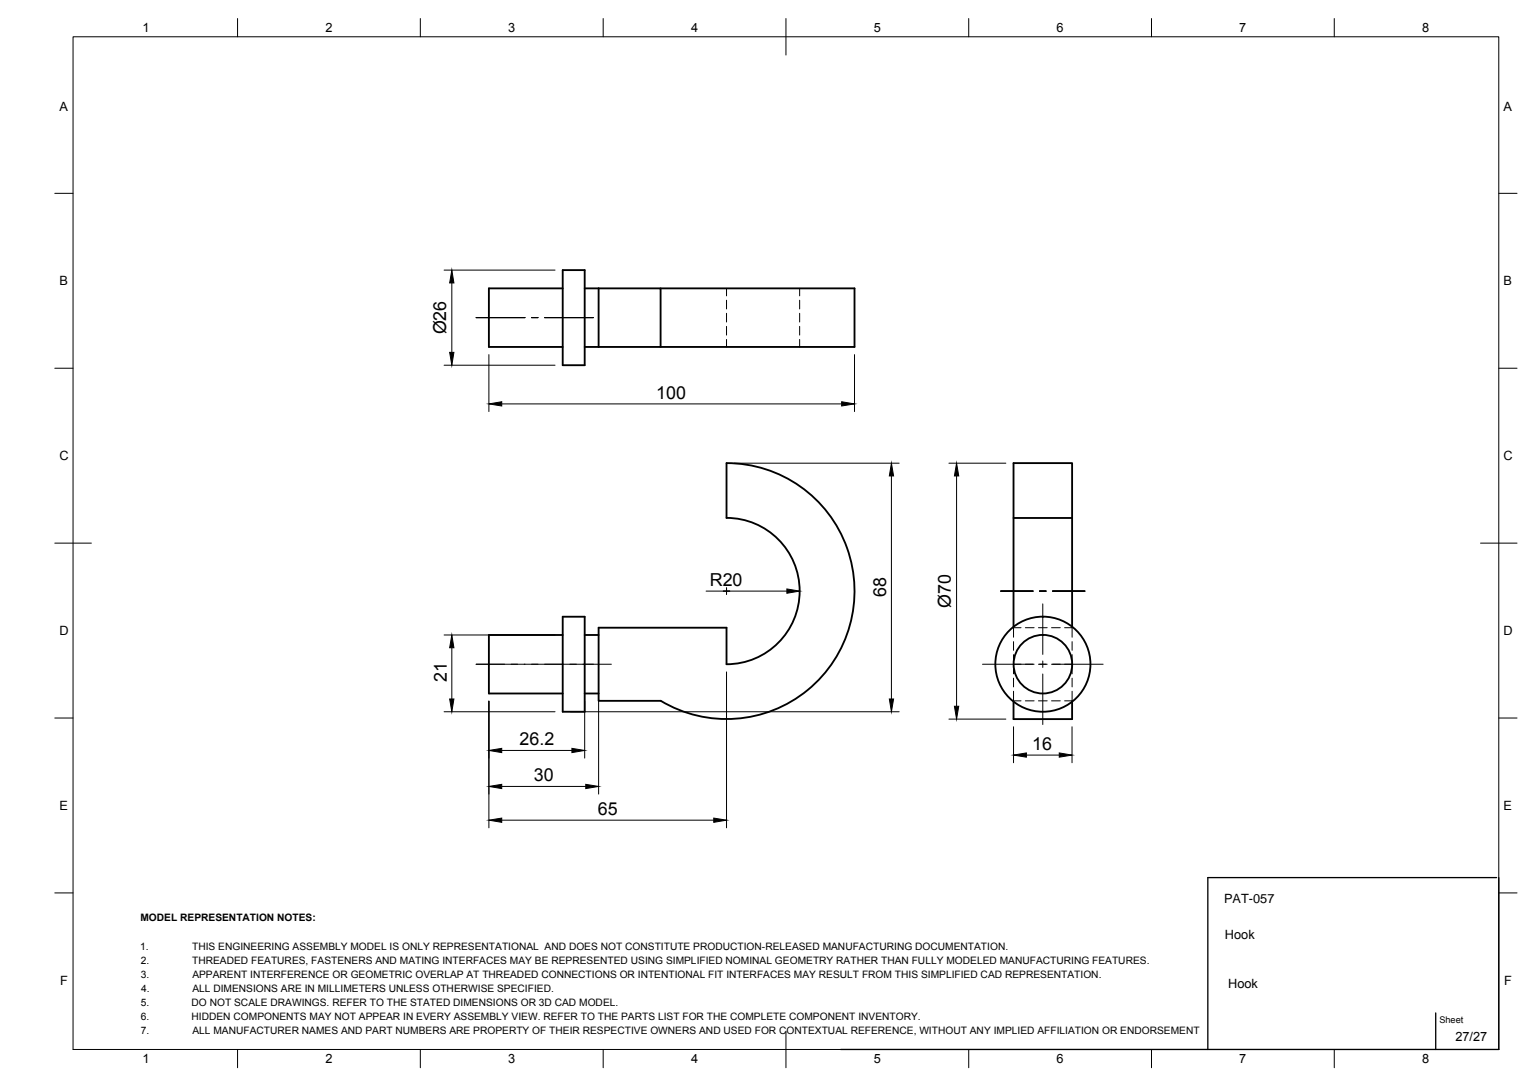
ISO-10303-21;
HEADER;
/* Generated by software containing ST-Developer
 * from STEP Tools, Inc. (www.steptools.com) 
 */

FILE_DESCRIPTION(
/* description */ ('Bearing-mounted hook block'),
/* implementation_level */ '2;1');

FILE_NAME(
/* name */ 'Hook.step',
/* time_stamp */ '2026-10-28T22:30:11-07:00',
/* author */ (''),
/* organization */ (''),
/* preprocessor_version */ 'ST-DEVELOPER v20.2',
/* originating_system */ 'Autodesk Translation Framework v15.17.0.0',
/* authorisation */ '');

FILE_SCHEMA (('AUTOMOTIVE_DESIGN { 1 0 10303 214 3 1 1 }'));
ENDSEC;

DATA;
#10=MECHANICAL_DESIGN_GEOMETRIC_PRESENTATION_REPRESENTATION('',(#352),#7609);
#296=SHAPE_REPRESENTATION_RELATIONSHIP('SRR','None',#7746,#320);
#320=ADVANCED_BREP_SHAPE_REPRESENTATION('',(#381),#7606);
#352=STYLED_ITEM('',(#7917),#381);
#381=MANIFOLD_SOLID_BREP('Body1',#3951);
#571=LINE('',#7423,#801);
#572=LINE('',#7426,#802);
#573=LINE('',#7435,#803);
#574=LINE('',#7439,#804);
#575=LINE('',#7441,#805);
#576=LINE('',#7442,#806);
#577=LINE('',#7445,#807);
#578=LINE('',#7447,#808);
#579=LINE('',#7448,#809);
#580=LINE('',#7452,#810);
#581=LINE('',#7453,#811);
#582=LINE('',#7454,#812);
#583=LINE('',#7458,#813);
#584=LINE('',#7460,#814);
#585=LINE('',#7462,#815);
#586=LINE('',#7463,#816);
#587=LINE('',#7465,#817);
#588=LINE('',#7469,#818);
#589=LINE('',#7474,#819);
#590=LINE('',#7476,#820);
#591=LINE('',#7479,#821);
#592=LINE('',#7482,#822);
#801=VECTOR('',#5924,1.3);
#802=VECTOR('',#5927,0.8);
#803=VECTOR('',#5938,0.8);
#804=VECTOR('',#5943,1.);
#805=VECTOR('',#5944,1.);
#806=VECTOR('',#5945,1.);
#807=VECTOR('',#5948,1.);
#808=VECTOR('',#5949,1.);
#809=VECTOR('',#5950,1.);
#810=VECTOR('',#5953,1.);
#811=VECTOR('',#5954,1.);
#812=VECTOR('',#5955,1.);
#813=VECTOR('',#5958,1.);
#814=VECTOR('',#5959,1.);
#815=VECTOR('',#5960,1.);
#816=VECTOR('',#5961,1.);
#817=VECTOR('',#5964,1.);
#818=VECTOR('',#5967,1.);
#819=VECTOR('',#5974,1.);
#820=VECTOR('',#5977,1.);
#821=VECTOR('',#5980,1.);
#822=VECTOR('',#5985,1.);
#913=CYLINDRICAL_SURFACE('',#4708,1.3);
#914=CYLINDRICAL_SURFACE('',#4709,0.8);
#915=CYLINDRICAL_SURFACE('',#4713,0.8);
#916=CYLINDRICAL_SURFACE('',#4723,2.);
#917=CYLINDRICAL_SURFACE('',#4729,3.5);
#995=FACE_BOUND('',#1519,.T.);
#996=FACE_BOUND('',#1521,.T.);
#1208=FACE_OUTER_BOUND('',#1518,.T.);
#1209=FACE_OUTER_BOUND('',#1520,.T.);
#1210=FACE_OUTER_BOUND('',#1522,.T.);
#1211=FACE_OUTER_BOUND('',#1523,.T.);
#1212=FACE_OUTER_BOUND('',#1524,.T.);
#1213=FACE_OUTER_BOUND('',#1525,.T.);
#1214=FACE_OUTER_BOUND('',#1526,.T.);
#1215=FACE_OUTER_BOUND('',#1527,.T.);
#1216=FACE_OUTER_BOUND('',#1528,.T.);
#1217=FACE_OUTER_BOUND('',#1529,.T.);
#1218=FACE_OUTER_BOUND('',#1530,.T.);
#1219=FACE_OUTER_BOUND('',#1531,.T.);
#1220=FACE_OUTER_BOUND('',#1532,.T.);
#1221=FACE_OUTER_BOUND('',#1533,.T.);
#1222=FACE_OUTER_BOUND('',#1534,.T.);
#1223=FACE_OUTER_BOUND('',#1535,.T.);
#1518=EDGE_LOOP('',(#3438));
#1519=EDGE_LOOP('',(#3439));
#1520=EDGE_LOOP('',(#3440));
#1521=EDGE_LOOP('',(#3441));
#1522=EDGE_LOOP('',(#3442,#3443,#3444,#3445));
#1523=EDGE_LOOP('',(#3446,#3447,#3448,#3449,#3450,#3451));
#1524=EDGE_LOOP('',(#3452,#3453,#3454,#3455));
#1525=EDGE_LOOP('',(#3456));
#1526=EDGE_LOOP('',(#3457,#3458,#3459,#3460));
#1527=EDGE_LOOP('',(#3461,#3462,#3463,#3464,#3465));
#1528=EDGE_LOOP('',(#3466,#3467,#3468,#3469));
#1529=EDGE_LOOP('',(#3470,#3471,#3472,#3473));
#1530=EDGE_LOOP('',(#3474,#3475,#3476,#3477,#3478,#3479,#3480,#3481));
#1531=EDGE_LOOP('',(#3482,#3483,#3484,#3485));
#1532=EDGE_LOOP('',(#3486,#3487,#3488,#3489,#3490,#3491,#3492,#3493));
#1533=EDGE_LOOP('',(#3494,#3495,#3496,#3497));
#1534=EDGE_LOOP('',(#3498,#3499,#3500,#3501));
#1535=EDGE_LOOP('',(#3502,#3503,#3504,#3505));
#1760=CIRCLE('',#4703,1.3);
#1761=CIRCLE('',#4704,0.8);
#1762=CIRCLE('',#4706,1.3);
#1763=CIRCLE('',#4707,0.8);
#1764=CIRCLE('',#4710,0.8);
#1765=CIRCLE('',#4711,0.8);
#1766=CIRCLE('',#4712,0.8);
#1767=CIRCLE('',#4714,0.8);
#1768=CIRCLE('',#4721,2.);
#1769=CIRCLE('',#4722,3.5);
#1770=CIRCLE('',#4724,2.);
#1771=CIRCLE('',#4726,3.5);
#2065=VERTEX_POINT('',#7413);
#2066=VERTEX_POINT('',#7415);
#2067=VERTEX_POINT('',#7418);
#2068=VERTEX_POINT('',#7420);
#2069=VERTEX_POINT('',#7425);
#2070=VERTEX_POINT('',#7427);
#2071=VERTEX_POINT('',#7429);
#2072=VERTEX_POINT('',#7433);
#2073=VERTEX_POINT('',#7438);
#2074=VERTEX_POINT('',#7440);
#2075=VERTEX_POINT('',#7444);
#2076=VERTEX_POINT('',#7446);
#2077=VERTEX_POINT('',#7450);
#2078=VERTEX_POINT('',#7451);
#2079=VERTEX_POINT('',#7456);
#2080=VERTEX_POINT('',#7457);
#2081=VERTEX_POINT('',#7459);
#2082=VERTEX_POINT('',#7461);
#2083=VERTEX_POINT('',#7466);
#2084=VERTEX_POINT('',#7468);
#2085=VERTEX_POINT('',#7472);
#2086=VERTEX_POINT('',#7477);
#2529=EDGE_CURVE('',#2065,#2065,#1760,.T.);
#2530=EDGE_CURVE('',#2066,#2066,#1761,.T.);
#2531=EDGE_CURVE('',#2067,#2067,#1762,.T.);
#2532=EDGE_CURVE('',#2068,#2068,#1763,.T.);
#2533=EDGE_CURVE('',#2065,#2067,#571,.T.);
#2534=EDGE_CURVE('',#2068,#2069,#572,.T.);
#2535=EDGE_CURVE('',#2070,#2069,#1764,.T.);
#2536=EDGE_CURVE('',#2071,#2070,#1765,.T.);
#2537=EDGE_CURVE('',#2069,#2071,#1766,.T.);
#2538=EDGE_CURVE('',#2072,#2072,#1767,.T.);
#2539=EDGE_CURVE('',#2072,#2066,#573,.T.);
#2540=EDGE_CURVE('',#2073,#2070,#574,.T.);
#2541=EDGE_CURVE('',#2073,#2074,#575,.T.);
#2542=EDGE_CURVE('',#2071,#2074,#576,.T.);
#2543=EDGE_CURVE('',#2075,#2071,#577,.T.);
#2544=EDGE_CURVE('',#2076,#2075,#578,.T.);
#2545=EDGE_CURVE('',#2070,#2076,#579,.T.);
#2546=EDGE_CURVE('',#2077,#2078,#580,.T.);
#2547=EDGE_CURVE('',#2076,#2077,#581,.T.);
#2548=EDGE_CURVE('',#2078,#2075,#582,.T.);
#2549=EDGE_CURVE('',#2079,#2080,#583,.T.);
#2550=EDGE_CURVE('',#2081,#2079,#584,.T.);
#2551=EDGE_CURVE('',#2082,#2081,#585,.T.);
#2552=EDGE_CURVE('',#2080,#2082,#586,.T.);
#2553=EDGE_CURVE('',#2074,#2081,#587,.T.);
#2554=EDGE_CURVE('',#2079,#2083,#1768,.T.);
#2555=EDGE_CURVE('',#2083,#2084,#588,.T.);
#2556=EDGE_CURVE('',#2084,#2078,#1769,.T.);
#2557=EDGE_CURVE('',#2080,#2085,#1770,.T.);
#2558=EDGE_CURVE('',#2085,#2083,#589,.T.);
#2559=EDGE_CURVE('',#2082,#2073,#590,.T.);
#2560=EDGE_CURVE('',#2086,#2077,#1771,.T.);
#2561=EDGE_CURVE('',#2086,#2085,#591,.T.);
#2562=EDGE_CURVE('',#2084,#2086,#592,.T.);
#3438=ORIENTED_EDGE('',*,*,#2529,.T.);
#3439=ORIENTED_EDGE('',*,*,#2530,.F.);
#3440=ORIENTED_EDGE('',*,*,#2531,.F.);
#3441=ORIENTED_EDGE('',*,*,#2532,.F.);
#3442=ORIENTED_EDGE('',*,*,#2529,.F.);
#3443=ORIENTED_EDGE('',*,*,#2533,.T.);
#3444=ORIENTED_EDGE('',*,*,#2531,.T.);
#3445=ORIENTED_EDGE('',*,*,#2533,.F.);
#3446=ORIENTED_EDGE('',*,*,#2532,.T.);
#3447=ORIENTED_EDGE('',*,*,#2534,.T.);
#3448=ORIENTED_EDGE('',*,*,#2535,.F.);
#3449=ORIENTED_EDGE('',*,*,#2536,.F.);
#3450=ORIENTED_EDGE('',*,*,#2537,.F.);
#3451=ORIENTED_EDGE('',*,*,#2534,.F.);
#3452=ORIENTED_EDGE('',*,*,#2538,.F.);
#3453=ORIENTED_EDGE('',*,*,#2539,.T.);
#3454=ORIENTED_EDGE('',*,*,#2530,.T.);
#3455=ORIENTED_EDGE('',*,*,#2539,.F.);
#3456=ORIENTED_EDGE('',*,*,#2538,.T.);
#3457=ORIENTED_EDGE('',*,*,#2536,.T.);
#3458=ORIENTED_EDGE('',*,*,#2540,.F.);
#3459=ORIENTED_EDGE('',*,*,#2541,.T.);
#3460=ORIENTED_EDGE('',*,*,#2542,.F.);
#3461=ORIENTED_EDGE('',*,*,#2535,.T.);
#3462=ORIENTED_EDGE('',*,*,#2537,.T.);
#3463=ORIENTED_EDGE('',*,*,#2543,.F.);
#3464=ORIENTED_EDGE('',*,*,#2544,.F.);
#3465=ORIENTED_EDGE('',*,*,#2545,.F.);
#3466=ORIENTED_EDGE('',*,*,#2546,.F.);
#3467=ORIENTED_EDGE('',*,*,#2547,.F.);
#3468=ORIENTED_EDGE('',*,*,#2544,.T.);
#3469=ORIENTED_EDGE('',*,*,#2548,.F.);
#3470=ORIENTED_EDGE('',*,*,#2549,.F.);
#3471=ORIENTED_EDGE('',*,*,#2550,.F.);
#3472=ORIENTED_EDGE('',*,*,#2551,.F.);
#3473=ORIENTED_EDGE('',*,*,#2552,.F.);
#3474=ORIENTED_EDGE('',*,*,#2553,.T.);
#3475=ORIENTED_EDGE('',*,*,#2550,.T.);
#3476=ORIENTED_EDGE('',*,*,#2554,.T.);
#3477=ORIENTED_EDGE('',*,*,#2555,.T.);
#3478=ORIENTED_EDGE('',*,*,#2556,.T.);
#3479=ORIENTED_EDGE('',*,*,#2548,.T.);
#3480=ORIENTED_EDGE('',*,*,#2543,.T.);
#3481=ORIENTED_EDGE('',*,*,#2542,.T.);
#3482=ORIENTED_EDGE('',*,*,#2549,.T.);
#3483=ORIENTED_EDGE('',*,*,#2557,.T.);
#3484=ORIENTED_EDGE('',*,*,#2558,.T.);
#3485=ORIENTED_EDGE('',*,*,#2554,.F.);
#3486=ORIENTED_EDGE('',*,*,#2559,.T.);
#3487=ORIENTED_EDGE('',*,*,#2540,.T.);
#3488=ORIENTED_EDGE('',*,*,#2545,.T.);
#3489=ORIENTED_EDGE('',*,*,#2547,.T.);
#3490=ORIENTED_EDGE('',*,*,#2560,.F.);
#3491=ORIENTED_EDGE('',*,*,#2561,.T.);
#3492=ORIENTED_EDGE('',*,*,#2557,.F.);
#3493=ORIENTED_EDGE('',*,*,#2552,.T.);
#3494=ORIENTED_EDGE('',*,*,#2559,.F.);
#3495=ORIENTED_EDGE('',*,*,#2551,.T.);
#3496=ORIENTED_EDGE('',*,*,#2553,.F.);
#3497=ORIENTED_EDGE('',*,*,#2541,.F.);
#3498=ORIENTED_EDGE('',*,*,#2562,.F.);
#3499=ORIENTED_EDGE('',*,*,#2555,.F.);
#3500=ORIENTED_EDGE('',*,*,#2558,.F.);
#3501=ORIENTED_EDGE('',*,*,#2561,.F.);
#3502=ORIENTED_EDGE('',*,*,#2546,.T.);
#3503=ORIENTED_EDGE('',*,*,#2556,.F.);
#3504=ORIENTED_EDGE('',*,*,#2562,.T.);
#3505=ORIENTED_EDGE('',*,*,#2560,.T.);
#3662=PLANE('',#4702);
#3663=PLANE('',#4705);
#3664=PLANE('',#4715);
#3665=PLANE('',#4716);
#3666=PLANE('',#4717);
#3667=PLANE('',#4718);
#3668=PLANE('',#4719);
#3669=PLANE('',#4720);
#3670=PLANE('',#4725);
#3671=PLANE('',#4727);
#3672=PLANE('',#4728);
#3890=ADVANCED_FACE('',(#1208,#995),#3662,.T.);
#3891=ADVANCED_FACE('',(#1209,#996),#3663,.F.);
#3892=ADVANCED_FACE('',(#1210),#913,.T.);
#3893=ADVANCED_FACE('',(#1211),#914,.T.);
#3894=ADVANCED_FACE('',(#1212),#915,.T.);
#3895=ADVANCED_FACE('',(#1213),#3664,.T.);
#3896=ADVANCED_FACE('',(#1214),#3665,.T.);
#3897=ADVANCED_FACE('',(#1215),#3666,.T.);
#3898=ADVANCED_FACE('',(#1216),#3667,.T.);
#3899=ADVANCED_FACE('',(#1217),#3668,.T.);
#3900=ADVANCED_FACE('',(#1218),#3669,.T.);
#3901=ADVANCED_FACE('',(#1219),#916,.F.);
#3902=ADVANCED_FACE('',(#1220),#3670,.F.);
#3903=ADVANCED_FACE('',(#1221),#3671,.F.);
#3904=ADVANCED_FACE('',(#1222),#3672,.F.);
#3905=ADVANCED_FACE('',(#1223),#917,.T.);
#3951=CLOSED_SHELL('',(#3890,#3891,#3892,#3893,#3894,#3895,#3896,#3897,
#3898,#3899,#3900,#3901,#3902,#3903,#3904,#3905));
#4701=AXIS2_PLACEMENT_3D('',#7411,#5908,#5909);
#4702=AXIS2_PLACEMENT_3D('',#7412,#5910,#5911);
#4703=AXIS2_PLACEMENT_3D('',#7414,#5912,#5913);
#4704=AXIS2_PLACEMENT_3D('',#7416,#5914,#5915);
#4705=AXIS2_PLACEMENT_3D('',#7417,#5916,#5917);
#4706=AXIS2_PLACEMENT_3D('',#7419,#5918,#5919);
#4707=AXIS2_PLACEMENT_3D('',#7421,#5920,#5921);
#4708=AXIS2_PLACEMENT_3D('',#7422,#5922,#5923);
#4709=AXIS2_PLACEMENT_3D('',#7424,#5925,#5926);
#4710=AXIS2_PLACEMENT_3D('',#7428,#5928,#5929);
#4711=AXIS2_PLACEMENT_3D('',#7430,#5930,#5931);
#4712=AXIS2_PLACEMENT_3D('',#7431,#5932,#5933);
#4713=AXIS2_PLACEMENT_3D('',#7432,#5934,#5935);
#4714=AXIS2_PLACEMENT_3D('',#7434,#5936,#5937);
#4715=AXIS2_PLACEMENT_3D('',#7436,#5939,#5940);
#4716=AXIS2_PLACEMENT_3D('',#7437,#5941,#5942);
#4717=AXIS2_PLACEMENT_3D('',#7443,#5946,#5947);
#4718=AXIS2_PLACEMENT_3D('',#7449,#5951,#5952);
#4719=AXIS2_PLACEMENT_3D('',#7455,#5956,#5957);
#4720=AXIS2_PLACEMENT_3D('',#7464,#5962,#5963);
#4721=AXIS2_PLACEMENT_3D('',#7467,#5965,#5966);
#4722=AXIS2_PLACEMENT_3D('',#7470,#5968,#5969);
#4723=AXIS2_PLACEMENT_3D('',#7471,#5970,#5971);
#4724=AXIS2_PLACEMENT_3D('',#7473,#5972,#5973);
#4725=AXIS2_PLACEMENT_3D('',#7475,#5975,#5976);
#4726=AXIS2_PLACEMENT_3D('',#7478,#5978,#5979);
#4727=AXIS2_PLACEMENT_3D('',#7480,#5981,#5982);
#4728=AXIS2_PLACEMENT_3D('',#7481,#5983,#5984);
#4729=AXIS2_PLACEMENT_3D('',#7483,#5986,#5987);
#5908=DIRECTION('axis',(0.,0.,1.));
#5909=DIRECTION('refdir',(1.,0.,0.));
#5910=DIRECTION('center_axis',(0.,0.,1.));
#5911=DIRECTION('ref_axis',(1.,0.,0.));
#5912=DIRECTION('center_axis',(0.,0.,1.));
#5913=DIRECTION('ref_axis',(1.,0.,0.));
#5914=DIRECTION('center_axis',(0.,0.,1.));
#5915=DIRECTION('ref_axis',(1.,0.,0.));
#5916=DIRECTION('center_axis',(0.,0.,1.));
#5917=DIRECTION('ref_axis',(1.,0.,0.));
#5918=DIRECTION('center_axis',(0.,0.,1.));
#5919=DIRECTION('ref_axis',(1.,0.,0.));
#5920=DIRECTION('center_axis',(0.,0.,-1.));
#5921=DIRECTION('ref_axis',(1.,0.,0.));
#5922=DIRECTION('center_axis',(0.,0.,1.));
#5923=DIRECTION('ref_axis',(1.,0.,0.));
#5924=DIRECTION('',(0.,0.,-1.));
#5925=DIRECTION('center_axis',(0.,0.,1.));
#5926=DIRECTION('ref_axis',(1.,0.,0.));
#5927=DIRECTION('',(0.,0.,-1.));
#5928=DIRECTION('center_axis',(0.,0.,-1.));
#5929=DIRECTION('ref_axis',(1.,0.,0.));
#5930=DIRECTION('center_axis',(0.,0.,-1.));
#5931=DIRECTION('ref_axis',(1.,0.,0.));
#5932=DIRECTION('center_axis',(0.,0.,-1.));
#5933=DIRECTION('ref_axis',(1.,0.,0.));
#5934=DIRECTION('center_axis',(0.,0.,1.));
#5935=DIRECTION('ref_axis',(1.,0.,0.));
#5936=DIRECTION('center_axis',(0.,0.,1.));
#5937=DIRECTION('ref_axis',(1.,0.,0.));
#5938=DIRECTION('',(0.,0.,-1.));
#5939=DIRECTION('center_axis',(0.,0.,1.));
#5940=DIRECTION('ref_axis',(1.,0.,0.));
#5941=DIRECTION('center_axis',(0.,0.,1.));
#5942=DIRECTION('ref_axis',(1.,0.,0.));
#5943=DIRECTION('',(-1.,0.,0.));
#5944=DIRECTION('',(0.,1.,0.));
#5945=DIRECTION('',(1.,0.,0.));
#5946=DIRECTION('center_axis',(0.,0.,1.));
#5947=DIRECTION('ref_axis',(1.,0.,0.));
#5948=DIRECTION('',(1.,0.,0.));
#5949=DIRECTION('',(0.,1.,0.));
#5950=DIRECTION('',(-1.,0.,0.));
#5951=DIRECTION('center_axis',(-1.,0.,0.));
#5952=DIRECTION('ref_axis',(0.,0.,1.));
#5953=DIRECTION('',(0.,1.,0.));
#5954=DIRECTION('',(0.,0.,-1.));
#5955=DIRECTION('',(0.,0.,1.));
#5956=DIRECTION('center_axis',(0.,0.,-1.));
#5957=DIRECTION('ref_axis',(-1.,0.,0.));
#5958=DIRECTION('',(0.,-1.,0.));
#5959=DIRECTION('',(-1.,0.,0.));
#5960=DIRECTION('',(0.,1.,0.));
#5961=DIRECTION('',(1.,0.,0.));
#5962=DIRECTION('center_axis',(0.,1.,0.));
#5963=DIRECTION('ref_axis',(1.,0.,0.));
#5964=DIRECTION('',(0.,0.,-1.));
#5965=DIRECTION('center_axis',(0.,-1.,0.));
#5966=DIRECTION('ref_axis',(1.,0.,0.));
#5967=DIRECTION('',(1.,0.,0.));
#5968=DIRECTION('center_axis',(0.,1.,0.));
#5969=DIRECTION('ref_axis',(1.,0.,0.));
#5970=DIRECTION('center_axis',(0.,1.,0.));
#5971=DIRECTION('ref_axis',(1.,0.,0.));
#5972=DIRECTION('center_axis',(0.,-1.,0.));
#5973=DIRECTION('ref_axis',(1.,0.,0.));
#5974=DIRECTION('',(0.,1.,0.));
#5975=DIRECTION('center_axis',(0.,1.,0.));
#5976=DIRECTION('ref_axis',(1.,0.,0.));
#5977=DIRECTION('',(0.,0.,1.));
#5978=DIRECTION('center_axis',(0.,1.,0.));
#5979=DIRECTION('ref_axis',(1.,0.,0.));
#5980=DIRECTION('',(-1.,0.,0.));
#5981=DIRECTION('center_axis',(-1.,0.,0.));
#5982=DIRECTION('ref_axis',(0.,0.,1.));
#5983=DIRECTION('center_axis',(0.,0.,-1.));
#5984=DIRECTION('ref_axis',(-1.,0.,0.));
#5985=DIRECTION('',(0.,-1.,0.));
#5986=DIRECTION('center_axis',(0.,1.,0.));
#5987=DIRECTION('ref_axis',(-0.267261241912424,0.,-0.963624111659432));
#7411=CARTESIAN_POINT('',(0.,0.,0.));
#7412=CARTESIAN_POINT('Origin',(0.,0.,4.48));
#7413=CARTESIAN_POINT('',(-1.3,-1.59204083889156E-16,4.48));
#7414=CARTESIAN_POINT('Origin',(0.,0.,4.48));
#7415=CARTESIAN_POINT('',(-0.8,-9.79717439317883E-17,4.48));
#7416=CARTESIAN_POINT('Origin',(0.,0.,4.48));
#7417=CARTESIAN_POINT('Origin',(0.,0.,3.88));
#7418=CARTESIAN_POINT('',(-1.3,-1.59204083889156E-16,3.88));
#7419=CARTESIAN_POINT('Origin',(0.,0.,3.88));
#7420=CARTESIAN_POINT('',(-0.8,9.79717439317883E-17,3.88));
#7421=CARTESIAN_POINT('Origin',(0.,0.,3.88));
#7422=CARTESIAN_POINT('Origin',(0.,0.,3.88));
#7423=CARTESIAN_POINT('',(-1.3,-1.59204083889156E-16,3.88));
#7424=CARTESIAN_POINT('Origin',(0.,0.,3.));
#7425=CARTESIAN_POINT('',(-0.8,-9.79717439317883E-17,3.5));
#7426=CARTESIAN_POINT('',(-0.8,-9.79717439317883E-17,3.));
#7427=CARTESIAN_POINT('',(0.,-0.8,3.5));
#7428=CARTESIAN_POINT('Origin',(0.,0.,3.5));
#7429=CARTESIAN_POINT('',(0.,0.8,3.5));
#7430=CARTESIAN_POINT('Origin',(0.,0.,3.5));
#7431=CARTESIAN_POINT('Origin',(0.,0.,3.5));
#7432=CARTESIAN_POINT('Origin',(0.,0.,3.));
#7433=CARTESIAN_POINT('',(-0.8,-9.79717439317883E-17,6.5));
#7434=CARTESIAN_POINT('Origin',(0.,0.,6.5));
#7435=CARTESIAN_POINT('',(-0.8,-9.79717439317883E-17,3.));
#7436=CARTESIAN_POINT('Origin',(0.,0.,6.5));
#7437=CARTESIAN_POINT('Origin',(-1.,-0.8,3.5));
#7438=CARTESIAN_POINT('',(1.,-0.8,3.5));
#7439=CARTESIAN_POINT('',(1.,-0.8,3.5));
#7440=CARTESIAN_POINT('',(1.,0.8,3.5));
#7441=CARTESIAN_POINT('',(1.,-0.8,3.5));
#7442=CARTESIAN_POINT('',(1.,0.8,3.5));
#7443=CARTESIAN_POINT('Origin',(-1.,-0.8,3.5));
#7444=CARTESIAN_POINT('',(-1.,0.8,3.5));
#7445=CARTESIAN_POINT('',(1.,0.8,3.5));
#7446=CARTESIAN_POINT('',(-1.,-0.8,3.5));
#7447=CARTESIAN_POINT('',(-1.,-0.8,3.5));
#7448=CARTESIAN_POINT('',(1.,-0.8,3.5));
#7449=CARTESIAN_POINT('Origin',(-1.,-0.8,0.));
#7450=CARTESIAN_POINT('',(-1.,-0.8,1.80277563773199));
#7451=CARTESIAN_POINT('',(-1.,0.8,1.80277563773199));
#7452=CARTESIAN_POINT('',(-1.,-0.8,1.80277563773199));
#7453=CARTESIAN_POINT('',(-1.,-0.8,3.5));
#7454=CARTESIAN_POINT('',(-1.,0.8,3.5));
#7455=CARTESIAN_POINT('Origin',(1.,-0.8,0.));
#7456=CARTESIAN_POINT('',(0.,0.8,0.));
#7457=CARTESIAN_POINT('',(0.,-0.8,0.));
#7458=CARTESIAN_POINT('',(0.,-0.8,0.));
#7459=CARTESIAN_POINT('',(1.,0.8,0.));
#7460=CARTESIAN_POINT('',(-1.,0.8,0.));
#7461=CARTESIAN_POINT('',(1.,-0.8,0.));
#7462=CARTESIAN_POINT('',(1.,-0.8,0.));
#7463=CARTESIAN_POINT('',(-1.,-0.8,0.));
#7464=CARTESIAN_POINT('Origin',(2.,0.8,0.));
#7465=CARTESIAN_POINT('',(1.,0.8,0.));
#7466=CARTESIAN_POINT('',(4.,0.8,0.));
#7467=CARTESIAN_POINT('Origin',(2.,0.8,0.));
#7468=CARTESIAN_POINT('',(5.5,0.8,0.));
#7469=CARTESIAN_POINT('',(4.,0.8,0.));
#7470=CARTESIAN_POINT('Origin',(2.,0.8,0.));
#7471=CARTESIAN_POINT('Origin',(2.,-0.8,0.));
#7472=CARTESIAN_POINT('',(4.,-0.8,0.));
#7473=CARTESIAN_POINT('Origin',(2.,-0.8,0.));
#7474=CARTESIAN_POINT('',(4.,-0.8,0.));
#7475=CARTESIAN_POINT('Origin',(2.,-0.8,0.));
#7476=CARTESIAN_POINT('',(1.,-0.8,0.));
#7477=CARTESIAN_POINT('',(5.5,-0.8,0.));
#7478=CARTESIAN_POINT('Origin',(2.,-0.8,0.));
#7479=CARTESIAN_POINT('',(4.,-0.8,0.));
#7480=CARTESIAN_POINT('Origin',(1.,-0.9,0.));
#7481=CARTESIAN_POINT('Origin',(6.,-0.9,0.));
#7482=CARTESIAN_POINT('',(5.5,-0.8,0.));
#7483=CARTESIAN_POINT('Origin',(2.,-0.8,0.));
#7576=UNCERTAINTY_MEASURE_WITH_UNIT(LENGTH_MEASURE(0.001),#7610,
'DISTANCE_ACCURACY_VALUE',
'Maximum model space distance between geometric entities at asserted c
onnectivities');
#7579=UNCERTAINTY_MEASURE_WITH_UNIT(LENGTH_MEASURE(0.001),#7610,
'DISTANCE_ACCURACY_VALUE',
'Maximum model space distance between geometric entities at asserted c
onnectivities');
#7606=(
GEOMETRIC_REPRESENTATION_CONTEXT(3)
GLOBAL_UNCERTAINTY_ASSIGNED_CONTEXT((#7576))
GLOBAL_UNIT_ASSIGNED_CONTEXT((#7610,#7612,#7613))
REPRESENTATION_CONTEXT('','3D')
);
#7609=(
GEOMETRIC_REPRESENTATION_CONTEXT(3)
GLOBAL_UNCERTAINTY_ASSIGNED_CONTEXT((#7579))
GLOBAL_UNIT_ASSIGNED_CONTEXT((#7610,#7612,#7613))
REPRESENTATION_CONTEXT('','3D')
);
#7610=(
LENGTH_UNIT()
NAMED_UNIT(*)
SI_UNIT(.CENTI.,.METRE.)
);
#7612=(
NAMED_UNIT(*)
PLANE_ANGLE_UNIT()
SI_UNIT($,.RADIAN.)
);
#7613=(
NAMED_UNIT(*)
SI_UNIT($,.STERADIAN.)
SOLID_ANGLE_UNIT()
);
#7640=SHAPE_DEFINITION_REPRESENTATION(#7711,#7746);
#7711=PRODUCT_DEFINITION_SHAPE('',$,#7776);
#7746=SHAPE_REPRESENTATION('',(#4701),#7606);
#7749=PRODUCT_DEFINITION_CONTEXT('part definition',#7838,'design');
#7776=PRODUCT_DEFINITION('Hook','Hook',#7805,#7749);
#7805=PRODUCT_DEFINITION_FORMATION('',$,#7866);
#7838=APPLICATION_CONTEXT(
'Core Data for Automotive Mechanical Design Process');
#7839=PRODUCT_CONTEXT('part definition',#7838,'mechanical');
#7866=PRODUCT('Hook','Hook','Hook',(#7839));
#7911=COLOUR_RGB('Light Blue',0.38,0.62,0.78);
#7912=FILL_AREA_STYLE_COLOUR('',#7911);
#7913=FILL_AREA_STYLE('',(#7912));
#7914=SURFACE_STYLE_FILL_AREA(#7913);
#7915=SURFACE_SIDE_STYLE('',(#7914));
#7916=SURFACE_STYLE_USAGE(.BOTH.,#7915);
#7917=PRESENTATION_STYLE_ASSIGNMENT((#7916));
ENDSEC;
END-ISO-10303-21;
